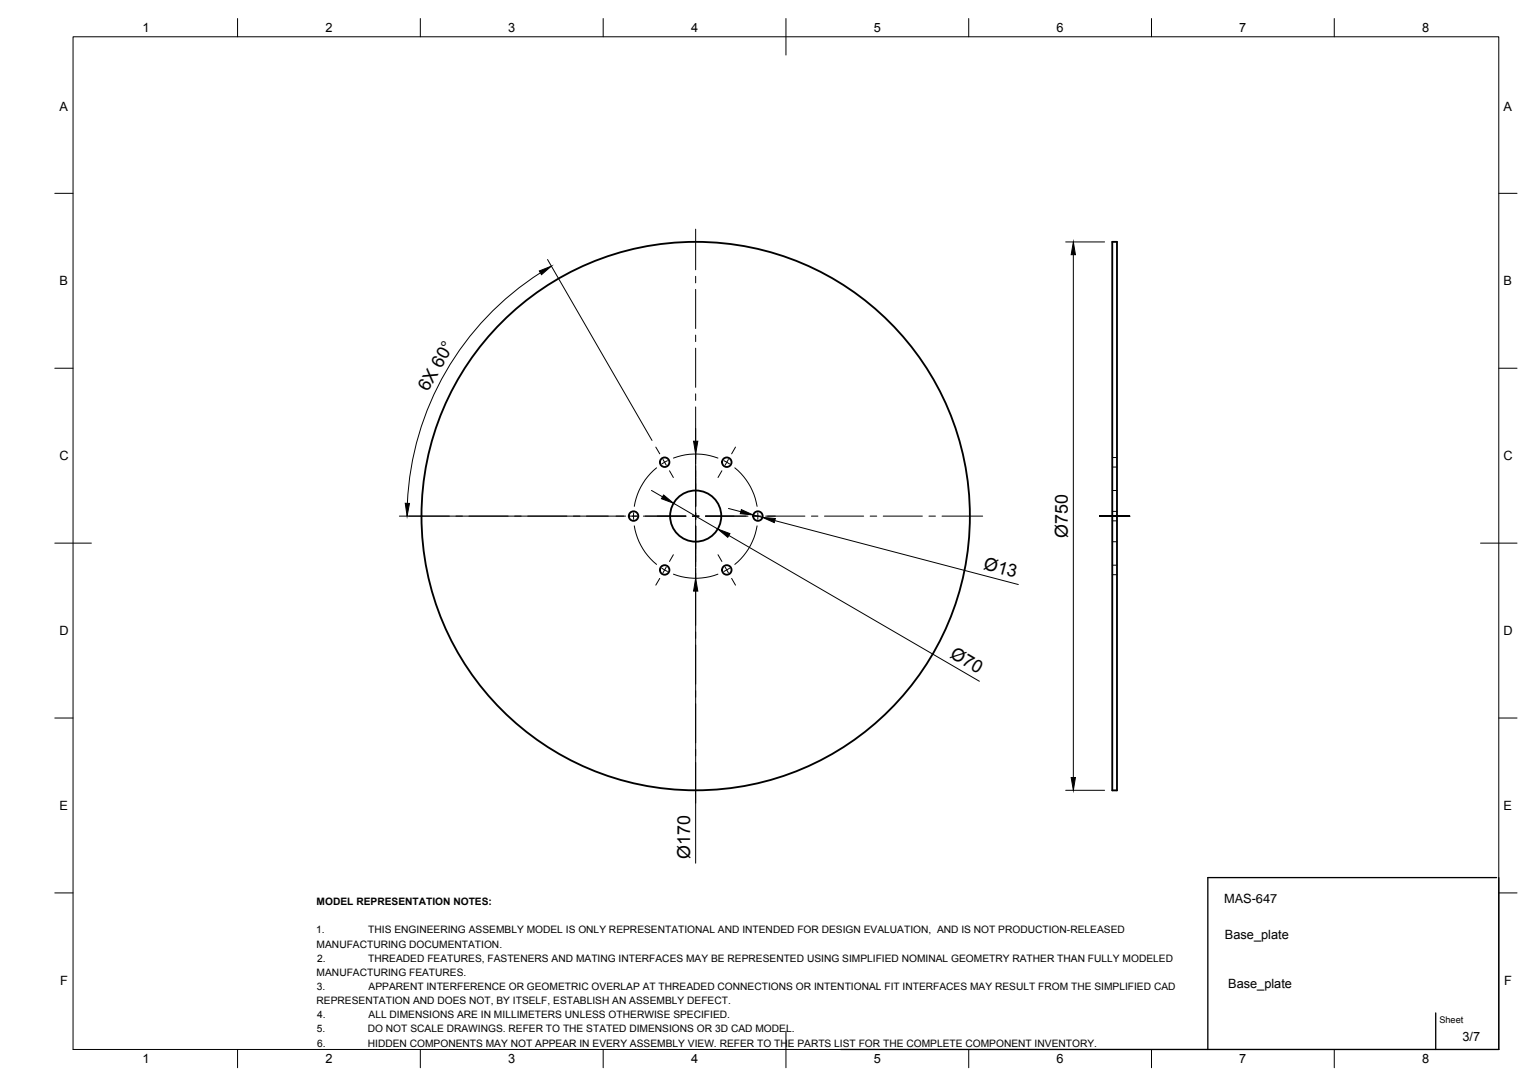
ISO-10303-21;
HEADER;
FILE_DESCRIPTION((''),'2;1');
FILE_NAME('Base_Plate.step','2026-10-09T11:36:02-07:00',(''),(''),'','','');
FILE_SCHEMA (('AUTOMOTIVE_DESIGN { 1 0 10303 214 3 1 1 }'));
ENDSEC;
DATA;
#10=MECHANICAL_DESIGN_GEOMETRIC_PRESENTATION_REPRESENTATION('',(#82),#1549);
#72=SHAPE_REPRESENTATION_RELATIONSHIP('SRR','None',#1581,#77) ;
#77=ADVANCED_BREP_SHAPE_REPRESENTATION('',(#87),#1544) ;
#82=STYLED_ITEM('',(#1615),#87) ;
#87=MANIFOLD_SOLID_BREP('Body1',#844) ;
#92=FACE_BOUND('',#196,.T.) ;
#93=FACE_BOUND('',#197,.T.) ;
#94=FACE_BOUND('',#198,.T.) ;
#95=FACE_BOUND('',#199,.T.) ;
#96=FACE_BOUND('',#200,.T.) ;
#97=FACE_BOUND('',#201,.T.) ;
#98=FACE_BOUND('',#202,.T.) ;
#99=FACE_BOUND('',#204,.T.) ;
#100=FACE_BOUND('',#205,.T.) ;
#101=FACE_BOUND('',#206,.T.) ;
#102=FACE_BOUND('',#207,.T.) ;
#103=FACE_BOUND('',#208,.T.) ;
#104=FACE_BOUND('',#209,.T.) ;
#105=FACE_BOUND('',#210,.T.) ;
#123=PLANE('',#931) ;
#124=PLANE('',#932) ;
#141=FACE_OUTER_BOUND('',#187,.T.) ;
#142=FACE_OUTER_BOUND('',#188,.T.) ;
#143=FACE_OUTER_BOUND('',#189,.T.) ;
#144=FACE_OUTER_BOUND('',#190,.T.) ;
#145=FACE_OUTER_BOUND('',#191,.T.) ;
#146=FACE_OUTER_BOUND('',#192,.T.) ;
#147=FACE_OUTER_BOUND('',#193,.T.) ;
#148=FACE_OUTER_BOUND('',#194,.T.) ;
#149=FACE_OUTER_BOUND('',#195,.T.) ;
#150=FACE_OUTER_BOUND('',#203,.T.) ;
#187=EDGE_LOOP('',(#575,#576,#577,#578)) ;
#188=EDGE_LOOP('',(#579,#580,#581,#582)) ;
#189=EDGE_LOOP('',(#583,#584,#585,#586)) ;
#190=EDGE_LOOP('',(#587,#588,#589,#590)) ;
#191=EDGE_LOOP('',(#591,#592,#593,#594)) ;
#192=EDGE_LOOP('',(#595,#596,#597,#598)) ;
#193=EDGE_LOOP('',(#599,#600,#601,#602)) ;
#194=EDGE_LOOP('',(#603,#604,#605,#606)) ;
#195=EDGE_LOOP('',(#607)) ;
#196=EDGE_LOOP('',(#608)) ;
#197=EDGE_LOOP('',(#609)) ;
#198=EDGE_LOOP('',(#610)) ;
#199=EDGE_LOOP('',(#611)) ;
#200=EDGE_LOOP('',(#612)) ;
#201=EDGE_LOOP('',(#613)) ;
#202=EDGE_LOOP('',(#614)) ;
#203=EDGE_LOOP('',(#615)) ;
#204=EDGE_LOOP('',(#616)) ;
#205=EDGE_LOOP('',(#617)) ;
#206=EDGE_LOOP('',(#618)) ;
#207=EDGE_LOOP('',(#619)) ;
#208=EDGE_LOOP('',(#620)) ;
#209=EDGE_LOOP('',(#621)) ;
#210=EDGE_LOOP('',(#622)) ;
#264=LINE('',#1313,#312) ;
#265=LINE('',#1319,#313) ;
#266=LINE('',#1325,#314) ;
#267=LINE('',#1331,#315) ;
#268=LINE('',#1337,#316) ;
#269=LINE('',#1343,#317) ;
#270=LINE('',#1349,#318) ;
#271=LINE('',#1355,#319) ;
#312=VECTOR('',#1031,6.49999999999999) ;
#313=VECTOR('',#1038,6.49999999999999) ;
#314=VECTOR('',#1045,6.49999999999999) ;
#315=VECTOR('',#1052,6.49999999999999) ;
#316=VECTOR('',#1059,6.49999999999999) ;
#317=VECTOR('',#1066,6.49999999999999) ;
#318=VECTOR('',#1073,35.) ;
#319=VECTOR('',#1080,375.) ;
#360=CIRCLE('',#908,6.49999999999999) ;
#361=CIRCLE('',#909,6.49999999999999) ;
#362=CIRCLE('',#911,6.49999999999999) ;
#363=CIRCLE('',#912,6.49999999999998) ;
#364=CIRCLE('',#914,6.49999999999999) ;
#365=CIRCLE('',#915,6.49999999999999) ;
#366=CIRCLE('',#917,6.49999999999999) ;
#367=CIRCLE('',#918,6.49999999999999) ;
#368=CIRCLE('',#920,6.49999999999999) ;
#369=CIRCLE('',#921,6.49999999999999) ;
#370=CIRCLE('',#923,6.49999999999999) ;
#371=CIRCLE('',#924,6.49999999999999) ;
#372=CIRCLE('',#926,35.) ;
#373=CIRCLE('',#927,35.) ;
#374=CIRCLE('',#929,375.) ;
#375=CIRCLE('',#930,375.) ;
#412=VERTEX_POINT('',#1310) ;
#413=VERTEX_POINT('',#1312) ;
#414=VERTEX_POINT('',#1316) ;
#415=VERTEX_POINT('',#1318) ;
#416=VERTEX_POINT('',#1322) ;
#417=VERTEX_POINT('',#1324) ;
#418=VERTEX_POINT('',#1328) ;
#419=VERTEX_POINT('',#1330) ;
#420=VERTEX_POINT('',#1334) ;
#421=VERTEX_POINT('',#1336) ;
#422=VERTEX_POINT('',#1340) ;
#423=VERTEX_POINT('',#1342) ;
#424=VERTEX_POINT('',#1346) ;
#425=VERTEX_POINT('',#1348) ;
#426=VERTEX_POINT('',#1352) ;
#427=VERTEX_POINT('',#1354) ;
#475=EDGE_CURVE('',#412,#412,#360,.T.) ;
#476=EDGE_CURVE('',#412,#413,#264,.T.) ;
#477=EDGE_CURVE('',#413,#413,#361,.T.) ;
#478=EDGE_CURVE('',#414,#414,#362,.T.) ;
#479=EDGE_CURVE('',#414,#415,#265,.T.) ;
#480=EDGE_CURVE('',#415,#415,#363,.T.) ;
#481=EDGE_CURVE('',#416,#416,#364,.T.) ;
#482=EDGE_CURVE('',#416,#417,#266,.T.) ;
#483=EDGE_CURVE('',#417,#417,#365,.T.) ;
#484=EDGE_CURVE('',#418,#418,#366,.T.) ;
#485=EDGE_CURVE('',#418,#419,#267,.T.) ;
#486=EDGE_CURVE('',#419,#419,#367,.T.) ;
#487=EDGE_CURVE('',#420,#420,#368,.T.) ;
#488=EDGE_CURVE('',#420,#421,#268,.T.) ;
#489=EDGE_CURVE('',#421,#421,#369,.T.) ;
#490=EDGE_CURVE('',#422,#422,#370,.T.) ;
#491=EDGE_CURVE('',#422,#423,#269,.T.) ;
#492=EDGE_CURVE('',#423,#423,#371,.T.) ;
#493=EDGE_CURVE('',#424,#424,#372,.T.) ;
#494=EDGE_CURVE('',#424,#425,#270,.T.) ;
#495=EDGE_CURVE('',#425,#425,#373,.T.) ;
#496=EDGE_CURVE('',#426,#426,#374,.T.) ;
#497=EDGE_CURVE('',#426,#427,#271,.T.) ;
#498=EDGE_CURVE('',#427,#427,#375,.T.) ;
#575=ORIENTED_EDGE('',*,*,#475,.F.) ;
#576=ORIENTED_EDGE('',*,*,#476,.T.) ;
#577=ORIENTED_EDGE('',*,*,#477,.T.) ;
#578=ORIENTED_EDGE('',*,*,#476,.F.) ;
#579=ORIENTED_EDGE('',*,*,#478,.F.) ;
#580=ORIENTED_EDGE('',*,*,#479,.T.) ;
#581=ORIENTED_EDGE('',*,*,#480,.T.) ;
#582=ORIENTED_EDGE('',*,*,#479,.F.) ;
#583=ORIENTED_EDGE('',*,*,#481,.F.) ;
#584=ORIENTED_EDGE('',*,*,#482,.T.) ;
#585=ORIENTED_EDGE('',*,*,#483,.T.) ;
#586=ORIENTED_EDGE('',*,*,#482,.F.) ;
#587=ORIENTED_EDGE('',*,*,#484,.F.) ;
#588=ORIENTED_EDGE('',*,*,#485,.T.) ;
#589=ORIENTED_EDGE('',*,*,#486,.T.) ;
#590=ORIENTED_EDGE('',*,*,#485,.F.) ;
#591=ORIENTED_EDGE('',*,*,#487,.F.) ;
#592=ORIENTED_EDGE('',*,*,#488,.T.) ;
#593=ORIENTED_EDGE('',*,*,#489,.T.) ;
#594=ORIENTED_EDGE('',*,*,#488,.F.) ;
#595=ORIENTED_EDGE('',*,*,#490,.F.) ;
#596=ORIENTED_EDGE('',*,*,#491,.T.) ;
#597=ORIENTED_EDGE('',*,*,#492,.T.) ;
#598=ORIENTED_EDGE('',*,*,#491,.F.) ;
#599=ORIENTED_EDGE('',*,*,#493,.F.) ;
#600=ORIENTED_EDGE('',*,*,#494,.T.) ;
#601=ORIENTED_EDGE('',*,*,#495,.T.) ;
#602=ORIENTED_EDGE('',*,*,#494,.F.) ;
#603=ORIENTED_EDGE('',*,*,#496,.F.) ;
#604=ORIENTED_EDGE('',*,*,#497,.T.) ;
#605=ORIENTED_EDGE('',*,*,#498,.T.) ;
#606=ORIENTED_EDGE('',*,*,#497,.F.) ;
#607=ORIENTED_EDGE('',*,*,#498,.F.) ;
#608=ORIENTED_EDGE('',*,*,#475,.T.) ;
#609=ORIENTED_EDGE('',*,*,#478,.T.) ;
#610=ORIENTED_EDGE('',*,*,#481,.T.) ;
#611=ORIENTED_EDGE('',*,*,#484,.T.) ;
#612=ORIENTED_EDGE('',*,*,#487,.T.) ;
#613=ORIENTED_EDGE('',*,*,#490,.T.) ;
#614=ORIENTED_EDGE('',*,*,#493,.T.) ;
#615=ORIENTED_EDGE('',*,*,#496,.T.) ;
#616=ORIENTED_EDGE('',*,*,#477,.F.) ;
#617=ORIENTED_EDGE('',*,*,#480,.F.) ;
#618=ORIENTED_EDGE('',*,*,#483,.F.) ;
#619=ORIENTED_EDGE('',*,*,#486,.F.) ;
#620=ORIENTED_EDGE('',*,*,#489,.F.) ;
#621=ORIENTED_EDGE('',*,*,#492,.F.) ;
#622=ORIENTED_EDGE('',*,*,#495,.F.) ;
#775=CYLINDRICAL_SURFACE('',#907,6.49999999999999) ;
#776=CYLINDRICAL_SURFACE('',#910,6.49999999999999) ;
#777=CYLINDRICAL_SURFACE('',#913,6.49999999999999) ;
#778=CYLINDRICAL_SURFACE('',#916,6.49999999999999) ;
#779=CYLINDRICAL_SURFACE('',#919,6.49999999999999) ;
#780=CYLINDRICAL_SURFACE('',#922,6.49999999999999) ;
#781=CYLINDRICAL_SURFACE('',#925,35.) ;
#782=CYLINDRICAL_SURFACE('',#928,375.) ;
#798=ADVANCED_FACE('',(#141),#775,.F.) ;
#799=ADVANCED_FACE('',(#142),#776,.F.) ;
#800=ADVANCED_FACE('',(#143),#777,.F.) ;
#801=ADVANCED_FACE('',(#144),#778,.F.) ;
#802=ADVANCED_FACE('',(#145),#779,.F.) ;
#803=ADVANCED_FACE('',(#146),#780,.F.) ;
#804=ADVANCED_FACE('',(#147),#781,.F.) ;
#805=ADVANCED_FACE('',(#148),#782,.T.) ;
#806=ADVANCED_FACE('',(#149,#92,#93,#94,#95,#96,#97,#98),#123,.F.) ;
#807=ADVANCED_FACE('',(#150,#99,#100,#101,#102,#103,#104,#105),#124,.T.) ;
#844=CLOSED_SHELL('',(#798,#799,#800,#801,#802,#803,#804,#805,#806,#807)) ;
#906=AXIS2_PLACEMENT_3D('',#1308,#1025,#1026) ;
#907=AXIS2_PLACEMENT_3D('',#1309,#1027,#1028) ;
#908=AXIS2_PLACEMENT_3D('',#1311,#1029,#1030) ;
#909=AXIS2_PLACEMENT_3D('',#1314,#1032,#1033) ;
#910=AXIS2_PLACEMENT_3D('',#1315,#1034,#1035) ;
#911=AXIS2_PLACEMENT_3D('',#1317,#1036,#1037) ;
#912=AXIS2_PLACEMENT_3D('',#1320,#1039,#1040) ;
#913=AXIS2_PLACEMENT_3D('',#1321,#1041,#1042) ;
#914=AXIS2_PLACEMENT_3D('',#1323,#1043,#1044) ;
#915=AXIS2_PLACEMENT_3D('',#1326,#1046,#1047) ;
#916=AXIS2_PLACEMENT_3D('',#1327,#1048,#1049) ;
#917=AXIS2_PLACEMENT_3D('',#1329,#1050,#1051) ;
#918=AXIS2_PLACEMENT_3D('',#1332,#1053,#1054) ;
#919=AXIS2_PLACEMENT_3D('',#1333,#1055,#1056) ;
#920=AXIS2_PLACEMENT_3D('',#1335,#1057,#1058) ;
#921=AXIS2_PLACEMENT_3D('',#1338,#1060,#1061) ;
#922=AXIS2_PLACEMENT_3D('',#1339,#1062,#1063) ;
#923=AXIS2_PLACEMENT_3D('',#1341,#1064,#1065) ;
#924=AXIS2_PLACEMENT_3D('',#1344,#1067,#1068) ;
#925=AXIS2_PLACEMENT_3D('',#1345,#1069,#1070) ;
#926=AXIS2_PLACEMENT_3D('',#1347,#1071,#1072) ;
#927=AXIS2_PLACEMENT_3D('',#1350,#1074,#1075) ;
#928=AXIS2_PLACEMENT_3D('',#1351,#1076,#1077) ;
#929=AXIS2_PLACEMENT_3D('',#1353,#1078,#1079) ;
#930=AXIS2_PLACEMENT_3D('',#1356,#1081,#1082) ;
#931=AXIS2_PLACEMENT_3D('',#1357,#1083,#1084) ;
#932=AXIS2_PLACEMENT_3D('',#1358,#1085,#1086) ;
#1025=DIRECTION('axis',(0.,0.,1.)) ;
#1026=DIRECTION('refdir',(1.,0.,0.)) ;
#1027=DIRECTION('center_axis',(1.,0.,0.)) ;
#1028=DIRECTION('ref_axis',(0.,0.,-1.)) ;
#1029=DIRECTION('center_axis',(1.,0.,0.)) ;
#1030=DIRECTION('ref_axis',(0.,0.,-1.)) ;
#1031=DIRECTION('',(1.,0.,0.)) ;
#1032=DIRECTION('center_axis',(1.,0.,0.)) ;
#1033=DIRECTION('ref_axis',(0.,0.,-1.)) ;
#1034=DIRECTION('center_axis',(1.,0.,0.)) ;
#1035=DIRECTION('ref_axis',(0.,0.,-1.)) ;
#1036=DIRECTION('center_axis',(1.,0.,0.)) ;
#1037=DIRECTION('ref_axis',(0.,0.,-1.)) ;
#1038=DIRECTION('',(1.,0.,0.)) ;
#1039=DIRECTION('center_axis',(1.,0.,0.)) ;
#1040=DIRECTION('ref_axis',(0.,0.,-1.)) ;
#1041=DIRECTION('center_axis',(1.,0.,0.)) ;
#1042=DIRECTION('ref_axis',(0.,0.,-1.)) ;
#1043=DIRECTION('center_axis',(1.,0.,0.)) ;
#1044=DIRECTION('ref_axis',(0.,0.,-1.)) ;
#1045=DIRECTION('',(1.,0.,0.)) ;
#1046=DIRECTION('center_axis',(1.,0.,0.)) ;
#1047=DIRECTION('ref_axis',(0.,0.,-1.)) ;
#1048=DIRECTION('center_axis',(1.,0.,0.)) ;
#1049=DIRECTION('ref_axis',(0.,0.,-1.)) ;
#1050=DIRECTION('center_axis',(1.,0.,0.)) ;
#1051=DIRECTION('ref_axis',(0.,0.,-1.)) ;
#1052=DIRECTION('',(1.,0.,0.)) ;
#1053=DIRECTION('center_axis',(1.,0.,0.)) ;
#1054=DIRECTION('ref_axis',(0.,0.,-1.)) ;
#1055=DIRECTION('center_axis',(1.,0.,0.)) ;
#1056=DIRECTION('ref_axis',(0.,0.,-1.)) ;
#1057=DIRECTION('center_axis',(1.,0.,0.)) ;
#1058=DIRECTION('ref_axis',(0.,0.,-1.)) ;
#1059=DIRECTION('',(1.,0.,0.)) ;
#1060=DIRECTION('center_axis',(1.,0.,0.)) ;
#1061=DIRECTION('ref_axis',(0.,0.,-1.)) ;
#1062=DIRECTION('center_axis',(1.,0.,0.)) ;
#1063=DIRECTION('ref_axis',(0.,0.,-1.)) ;
#1064=DIRECTION('center_axis',(1.,0.,0.)) ;
#1065=DIRECTION('ref_axis',(0.,0.,-1.)) ;
#1066=DIRECTION('',(1.,0.,0.)) ;
#1067=DIRECTION('center_axis',(1.,0.,0.)) ;
#1068=DIRECTION('ref_axis',(0.,0.,-1.)) ;
#1069=DIRECTION('center_axis',(1.,0.,0.)) ;
#1070=DIRECTION('ref_axis',(0.,0.,-1.)) ;
#1071=DIRECTION('center_axis',(1.,0.,0.)) ;
#1072=DIRECTION('ref_axis',(0.,0.,-1.)) ;
#1073=DIRECTION('',(1.,0.,0.)) ;
#1074=DIRECTION('center_axis',(1.,0.,0.)) ;
#1075=DIRECTION('ref_axis',(0.,0.,-1.)) ;
#1076=DIRECTION('center_axis',(1.,0.,0.)) ;
#1077=DIRECTION('ref_axis',(0.,0.,-1.)) ;
#1078=DIRECTION('center_axis',(1.,0.,0.)) ;
#1079=DIRECTION('ref_axis',(0.,0.,-1.)) ;
#1080=DIRECTION('',(-1.,0.,0.)) ;
#1081=DIRECTION('center_axis',(1.,0.,0.)) ;
#1082=DIRECTION('ref_axis',(0.,0.,-1.)) ;
#1083=DIRECTION('center_axis',(1.,0.,0.)) ;
#1084=DIRECTION('ref_axis',(0.,0.,-1.)) ;
#1085=DIRECTION('center_axis',(1.,0.,0.)) ;
#1086=DIRECTION('ref_axis',(0.,0.,-1.)) ;
#1308=CARTESIAN_POINT('',(0.,0.,0.)) ;
#1309=CARTESIAN_POINT('Origin',(0.,42.5000000000009,73.6121593216768)) ;
#1310=CARTESIAN_POINT('',(-6.35,42.5000000000009,80.1121593216768)) ;
#1311=CARTESIAN_POINT('Origin',(-6.35,42.5000000000009,73.6121593216768)) ;
#1312=CARTESIAN_POINT('',(7.59281015471356E-16,42.5000000000009,80.1121593216768)) ;
#1313=CARTESIAN_POINT('',(0.,42.5000000000009,80.1121593216768)) ;
#1314=CARTESIAN_POINT('Origin',(7.59281015471356E-16,42.5000000000009,73.6121593216768)) ;
#1315=CARTESIAN_POINT('Origin',(0.,-42.4999999999993,73.6121593216777)) ;
#1316=CARTESIAN_POINT('',(-6.35,-42.4999999999993,80.1121593216777)) ;
#1317=CARTESIAN_POINT('Origin',(-6.35,-42.4999999999993,73.6121593216777)) ;
#1318=CARTESIAN_POINT('',(7.59281015471356E-16,-42.4999999999993,80.1121593216777)) ;
#1319=CARTESIAN_POINT('',(0.,-42.4999999999993,80.1121593216777)) ;
#1320=CARTESIAN_POINT('Origin',(7.59281015471356E-16,-42.4999999999993,
73.6121593216777)) ;
#1321=CARTESIAN_POINT('Origin',(0.,-85.,0.)) ;
#1322=CARTESIAN_POINT('',(-6.35,-85.,6.49999999999999)) ;
#1323=CARTESIAN_POINT('Origin',(-6.35,-85.,0.)) ;
#1324=CARTESIAN_POINT('',(7.59281015471356E-16,-85.,6.49999999999999)) ;
#1325=CARTESIAN_POINT('',(0.,-85.,6.49999999999999)) ;
#1326=CARTESIAN_POINT('Origin',(7.59281015471356E-16,-85.,0.)) ;
#1327=CARTESIAN_POINT('Origin',(0.,-42.5000000000004,-73.6121593216771)) ;
#1328=CARTESIAN_POINT('',(-6.35,-42.5000000000004,-67.1121593216771)) ;
#1329=CARTESIAN_POINT('Origin',(-6.35,-42.5000000000004,-73.6121593216771)) ;
#1330=CARTESIAN_POINT('',(7.59281015471356E-16,-42.5000000000004,-67.1121593216771)) ;
#1331=CARTESIAN_POINT('',(0.,-42.5000000000004,-67.1121593216771)) ;
#1332=CARTESIAN_POINT('Origin',(7.59281015471356E-16,-42.5000000000004,
-73.6121593216771)) ;
#1333=CARTESIAN_POINT('Origin',(0.,42.4999999999999,-73.6121593216774)) ;
#1334=CARTESIAN_POINT('',(-6.35,42.4999999999999,-67.1121593216774)) ;
#1335=CARTESIAN_POINT('Origin',(-6.35,42.4999999999999,-73.6121593216774)) ;
#1336=CARTESIAN_POINT('',(7.59281015471356E-16,42.4999999999999,-67.1121593216774)) ;
#1337=CARTESIAN_POINT('',(0.,42.4999999999999,-67.1121593216774)) ;
#1338=CARTESIAN_POINT('Origin',(7.59281015471356E-16,42.4999999999999,-73.6121593216774)) ;
#1339=CARTESIAN_POINT('Origin',(0.,85.,0.)) ;
#1340=CARTESIAN_POINT('',(-6.35,85.,6.49999999999999)) ;
#1341=CARTESIAN_POINT('Origin',(-6.35,85.,0.)) ;
#1342=CARTESIAN_POINT('',(7.59281015471356E-16,85.,6.49999999999999)) ;
#1343=CARTESIAN_POINT('',(0.,85.,6.49999999999999)) ;
#1344=CARTESIAN_POINT('Origin',(7.59281015471356E-16,85.,0.)) ;
#1345=CARTESIAN_POINT('Origin',(-6.35,0.,0.)) ;
#1346=CARTESIAN_POINT('',(-6.35,-4.28626379701574E-15,35.)) ;
#1347=CARTESIAN_POINT('Origin',(-6.35,0.,0.)) ;
#1348=CARTESIAN_POINT('',(0.,-4.28626379701574E-15,35.)) ;
#1349=CARTESIAN_POINT('',(-6.35,-4.28626379701574E-15,35.)) ;
#1350=CARTESIAN_POINT('Origin',(0.,0.,0.)) ;
#1351=CARTESIAN_POINT('Origin',(-6.35,0.,0.)) ;
#1352=CARTESIAN_POINT('',(1.11022302462516E-15,-4.59242549680257E-14,375.)) ;
#1353=CARTESIAN_POINT('Origin',(0.,0.,0.)) ;
#1354=CARTESIAN_POINT('',(-6.35,-4.59242549680257E-14,375.)) ;
#1355=CARTESIAN_POINT('',(-6.35,-4.59242549680257E-14,375.)) ;
#1356=CARTESIAN_POINT('Origin',(-6.35,0.,0.)) ;
#1357=CARTESIAN_POINT('Origin',(-6.35,0.,0.)) ;
#1358=CARTESIAN_POINT('Origin',(0.,0.,0.)) ;
#1537=UNCERTAINTY_MEASURE_WITH_UNIT(LENGTH_MEASURE(0.01),#1550,
'DISTANCE_ACCURACY_VALUE',
'Maximum model space distance between geometric entities at asserted c
onnectivities') ;
#1542=UNCERTAINTY_MEASURE_WITH_UNIT(LENGTH_MEASURE(0.01),#1550,
'DISTANCE_ACCURACY_VALUE',
'Maximum model space distance between geometric entities at asserted c
onnectivities') ;
#1544=(
GEOMETRIC_REPRESENTATION_CONTEXT(3)
GLOBAL_UNCERTAINTY_ASSIGNED_CONTEXT((#1537))
GLOBAL_UNIT_ASSIGNED_CONTEXT((#1550,#1552,#1553))
REPRESENTATION_CONTEXT('','3D')
) ;
#1549=(
GEOMETRIC_REPRESENTATION_CONTEXT(3)
GLOBAL_UNCERTAINTY_ASSIGNED_CONTEXT((#1542))
GLOBAL_UNIT_ASSIGNED_CONTEXT((#1550,#1552,#1553))
REPRESENTATION_CONTEXT('','3D')
) ;
#1550=(
LENGTH_UNIT()
NAMED_UNIT(*)
SI_UNIT(.MILLI.,.METRE.)
) ;
#1552=(
NAMED_UNIT(*)
PLANE_ANGLE_UNIT()
SI_UNIT($,.RADIAN.)
) ;
#1553=(
NAMED_UNIT(*)
SI_UNIT($,.STERADIAN.)
SOLID_ANGLE_UNIT()
) ;
#1555=SHAPE_DEFINITION_REPRESENTATION(#1561,#1581) ;
#1561=PRODUCT_DEFINITION_SHAPE('',$,#1588) ;
#1581=SHAPE_REPRESENTATION('',(#906),#1544) ;
#1586=PRODUCT_DEFINITION_CONTEXT('part definition',#1606,'design') ;
#1588=PRODUCT_DEFINITION('Base_Plate','Base_Plate',#1594,#1586) ;
#1594=PRODUCT_DEFINITION_FORMATION('',$,#1609) ;
#1606=APPLICATION_CONTEXT(
'Core Data for Automotive Mechanical Design Process') ;
#1607=PRODUCT_CONTEXT('part definition',#1606,'mechanical') ;
#1609=PRODUCT('Base_Plate','Base_Plate',$,(#1607)) ;
#1615=PRESENTATION_STYLE_ASSIGNMENT((#1617)) ;
#1617=SURFACE_STYLE_USAGE(.BOTH.,#1619) ;
#1619=SURFACE_SIDE_STYLE('',(#1621)) ;
#1621=SURFACE_STYLE_FILL_AREA(#1623) ;
#1623=FILL_AREA_STYLE('Opaque(202,209,238)',(#1625)) ;
#1625=FILL_AREA_STYLE_COLOUR('Opaque(202,209,238)',#1627) ;
#1627=COLOUR_RGB('Opaque(202,209,238)', 0.09019608, 0.27058824, 0.51372549) ;
ENDSEC;
END-ISO-10303-21;
